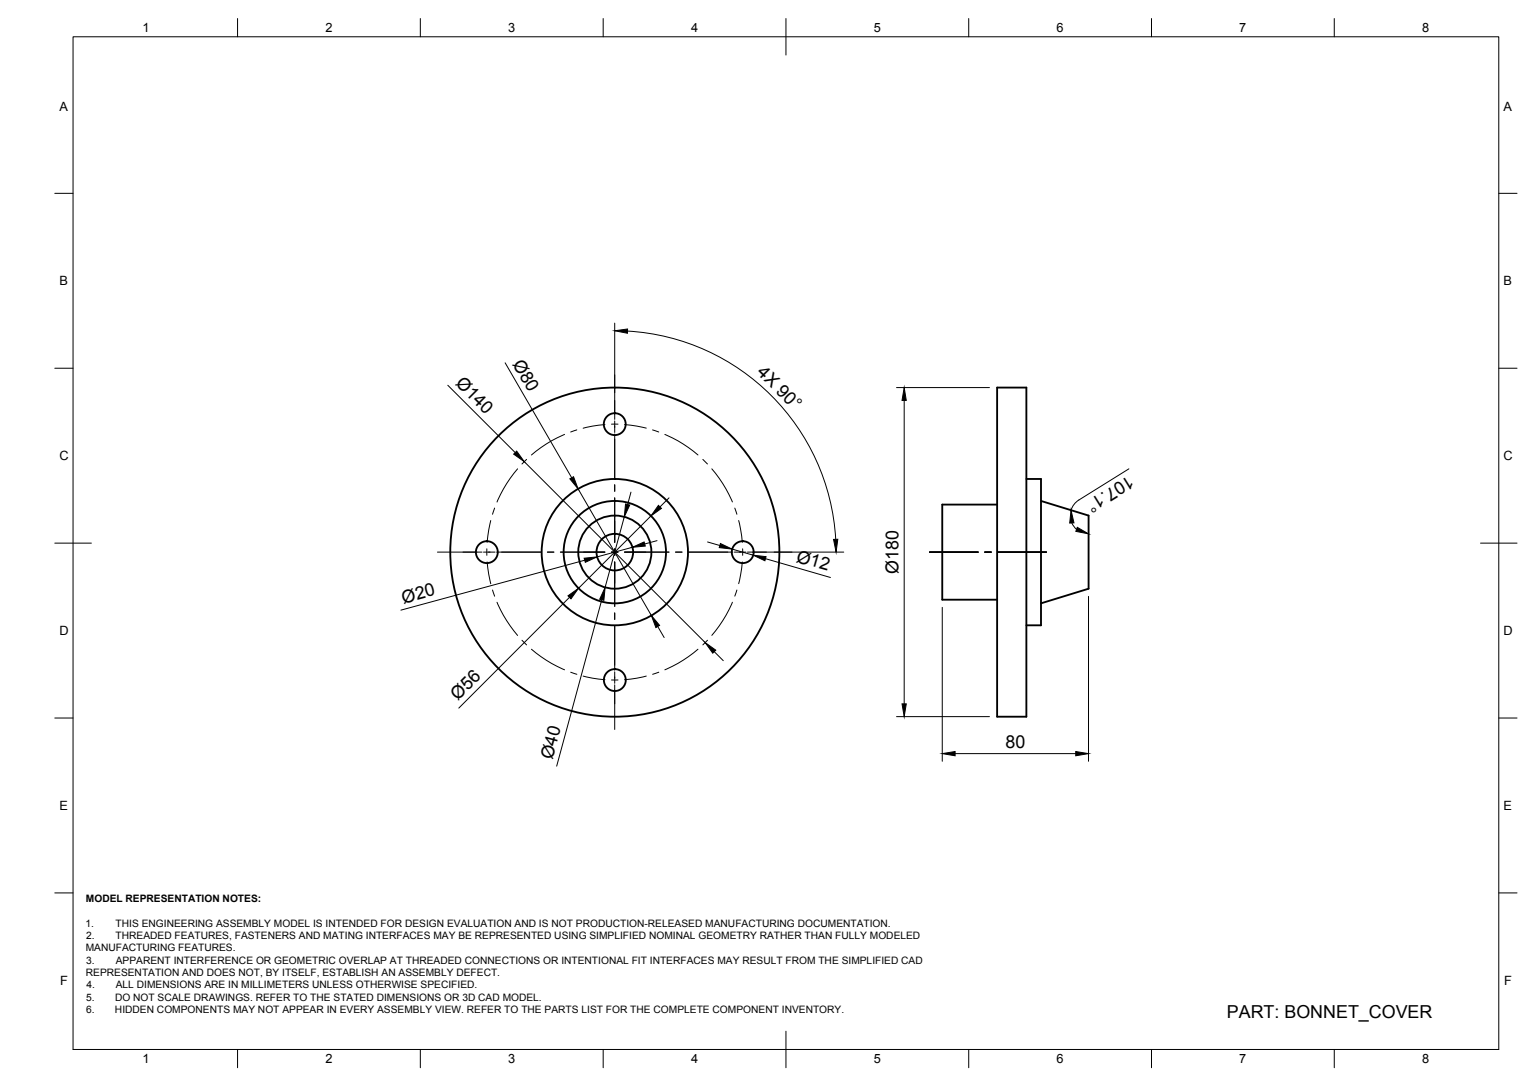
ISO-10303-21;
HEADER;
/* Generated by software containing ST-Developer
 * from STEP Tools, Inc. (www.steptools.com) 
 */

FILE_DESCRIPTION(
/* description */ (''),
/* implementation_level */ '2;1');

FILE_NAME(
/* name */ 'BONNET_COVER.step',
/* time_stamp */ '2026-10-04T02:10:06-07:00',
/* author */ (''),
/* organization */ (''),
/* preprocessor_version */ 'ST-DEVELOPER v20.2',
/* originating_system */ 'Autodesk Translation Framework v15.15.0.0',
/* authorisation */ '');

FILE_SCHEMA (('AUTOMOTIVE_DESIGN { 1 0 10303 214 3 1 1 }'));
ENDSEC;

DATA;
#10=MECHANICAL_DESIGN_GEOMETRIC_PRESENTATION_REPRESENTATION('',(#146),#9668);
#124=SHAPE_REPRESENTATION_RELATIONSHIP('SRR','None',#9717,#135);
#135=ADVANCED_BREP_SHAPE_REPRESENTATION('',(#157),#9662);
#146=STYLED_ITEM('',(#9775),#157);
#157=MANIFOLD_SOLID_BREP('Body1',#3886);
#173=CONICAL_SURFACE('',#4247,18.,1.1071487177941);
#174=CONICAL_SURFACE('',#4254,19.9999999999999,0.298498931586182);
#241=FACE_BOUND('',#1184,.T.);
#242=FACE_BOUND('',#1189,.T.);
#243=FACE_BOUND('',#1192,.T.);
#244=FACE_BOUND('',#1195,.T.);
#245=FACE_BOUND('',#1196,.T.);
#246=FACE_BOUND('',#1197,.T.);
#247=FACE_BOUND('',#1198,.T.);
#248=FACE_BOUND('',#1199,.T.);
#249=FACE_BOUND('',#1202,.T.);
#250=FACE_BOUND('',#1203,.T.);
#251=FACE_BOUND('',#1204,.T.);
#252=FACE_BOUND('',#1205,.T.);
#253=FACE_BOUND('',#1206,.T.);
#315=PLANE('',#4241);
#316=PLANE('',#4252);
#317=PLANE('',#4256);
#318=PLANE('',#4260);
#319=PLANE('',#4268);
#473=LINE('',#6782,#664);
#474=LINE('',#6791,#665);
#475=LINE('',#6794,#666);
#476=LINE('',#6802,#667);
#477=LINE('',#6808,#668);
#478=LINE('',#6823,#669);
#479=LINE('',#6837,#670);
#480=LINE('',#6839,#671);
#481=LINE('',#6841,#672);
#482=LINE('',#6843,#673);
#483=LINE('',#6845,#674);
#664=VECTOR('',#5033,18.0000000000001);
#665=VECTOR('',#5044,18.);
#666=VECTOR('',#5047,9.99999999999995);
#667=VECTOR('',#5058,19.9999999999999);
#668=VECTOR('',#5065,40.);
#669=VECTOR('',#5082,89.999999999998);
#670=VECTOR('',#5099,25.999999999998);
#671=VECTOR('',#5102,6.);
#672=VECTOR('',#5105,6.);
#673=VECTOR('',#5108,6.);
#674=VECTOR('',#5111,6.);
#792=CYLINDRICAL_SURFACE('',#4244,18.0000000000001);
#793=CYLINDRICAL_SURFACE('',#4250,9.99999999999995);
#794=CYLINDRICAL_SURFACE('',#4258,40.);
#795=CYLINDRICAL_SURFACE('',#4266,89.999999999998);
#796=CYLINDRICAL_SURFACE('',#4274,25.999999999998);
#797=CYLINDRICAL_SURFACE('',#4275,6.);
#798=CYLINDRICAL_SURFACE('',#4276,6.);
#799=CYLINDRICAL_SURFACE('',#4277,6.);
#800=CYLINDRICAL_SURFACE('',#4278,6.);
#914=FACE_OUTER_BOUND('',#1183,.T.);
#915=FACE_OUTER_BOUND('',#1185,.T.);
#916=FACE_OUTER_BOUND('',#1186,.T.);
#917=FACE_OUTER_BOUND('',#1187,.T.);
#918=FACE_OUTER_BOUND('',#1188,.T.);
#919=FACE_OUTER_BOUND('',#1190,.T.);
#920=FACE_OUTER_BOUND('',#1191,.T.);
#921=FACE_OUTER_BOUND('',#1193,.T.);
#922=FACE_OUTER_BOUND('',#1194,.T.);
#923=FACE_OUTER_BOUND('',#1200,.T.);
#924=FACE_OUTER_BOUND('',#1201,.T.);
#925=FACE_OUTER_BOUND('',#1207,.T.);
#926=FACE_OUTER_BOUND('',#1208,.T.);
#927=FACE_OUTER_BOUND('',#1209,.T.);
#928=FACE_OUTER_BOUND('',#1210,.T.);
#929=FACE_OUTER_BOUND('',#1211,.T.);
#1183=EDGE_LOOP('',(#3053));
#1184=EDGE_LOOP('',(#3054));
#1185=EDGE_LOOP('',(#3055,#3056,#3057,#3058,#3059));
#1186=EDGE_LOOP('',(#3060,#3061,#3062,#3063,#3064,#3065));
#1187=EDGE_LOOP('',(#3066,#3067,#3068,#3069,#3070));
#1188=EDGE_LOOP('',(#3071));
#1189=EDGE_LOOP('',(#3072));
#1190=EDGE_LOOP('',(#3073,#3074,#3075,#3076));
#1191=EDGE_LOOP('',(#3077));
#1192=EDGE_LOOP('',(#3078));
#1193=EDGE_LOOP('',(#3079,#3080,#3081,#3082));
#1194=EDGE_LOOP('',(#3083));
#1195=EDGE_LOOP('',(#3084));
#1196=EDGE_LOOP('',(#3085));
#1197=EDGE_LOOP('',(#3086));
#1198=EDGE_LOOP('',(#3087));
#1199=EDGE_LOOP('',(#3088));
#1200=EDGE_LOOP('',(#3089,#3090,#3091,#3092));
#1201=EDGE_LOOP('',(#3093));
#1202=EDGE_LOOP('',(#3094));
#1203=EDGE_LOOP('',(#3095));
#1204=EDGE_LOOP('',(#3096));
#1205=EDGE_LOOP('',(#3097));
#1206=EDGE_LOOP('',(#3098));
#1207=EDGE_LOOP('',(#3099,#3100,#3101,#3102));
#1208=EDGE_LOOP('',(#3103,#3104,#3105,#3106));
#1209=EDGE_LOOP('',(#3107,#3108,#3109,#3110));
#1210=EDGE_LOOP('',(#3111,#3112,#3113,#3114));
#1211=EDGE_LOOP('',(#3115,#3116,#3117,#3118));
#1543=CIRCLE('',#4242,25.999999999998);
#1544=CIRCLE('',#4243,18.0000000000002);
#1545=CIRCLE('',#4245,18.);
#1546=CIRCLE('',#4246,18.);
#1547=CIRCLE('',#4248,10.);
#1548=CIRCLE('',#4249,10.);
#1549=CIRCLE('',#4251,9.9999999999999);
#1550=CIRCLE('',#4253,19.9999999999999);
#1551=CIRCLE('',#4255,28.);
#1552=CIRCLE('',#4257,40.);
#1553=CIRCLE('',#4259,40.);
#1554=CIRCLE('',#4261,89.999999999998);
#1555=CIRCLE('',#4262,6.);
#1556=CIRCLE('',#4263,6.);
#1557=CIRCLE('',#4264,6.);
#1558=CIRCLE('',#4265,6.);
#1559=CIRCLE('',#4267,89.999999999998);
#1560=CIRCLE('',#4269,6.);
#1561=CIRCLE('',#4270,6.);
#1562=CIRCLE('',#4271,6.);
#1563=CIRCLE('',#4272,6.);
#1564=CIRCLE('',#4273,25.9999999999979);
#1809=VERTEX_POINT('',#6776);
#1810=VERTEX_POINT('',#6778);
#1811=VERTEX_POINT('',#6781);
#1812=VERTEX_POINT('',#6783);
#1813=VERTEX_POINT('',#6787);
#1814=VERTEX_POINT('',#6788);
#1815=VERTEX_POINT('',#6793);
#1816=VERTEX_POINT('',#6797);
#1817=VERTEX_POINT('',#6800);
#1818=VERTEX_POINT('',#6804);
#1819=VERTEX_POINT('',#6807);
#1820=VERTEX_POINT('',#6811);
#1821=VERTEX_POINT('',#6813);
#1822=VERTEX_POINT('',#6815);
#1823=VERTEX_POINT('',#6817);
#1824=VERTEX_POINT('',#6819);
#1825=VERTEX_POINT('',#6822);
#1826=VERTEX_POINT('',#6826);
#1827=VERTEX_POINT('',#6828);
#1828=VERTEX_POINT('',#6830);
#1829=VERTEX_POINT('',#6832);
#1830=VERTEX_POINT('',#6834);
#2250=EDGE_CURVE('',#1809,#1809,#1543,.T.);
#2251=EDGE_CURVE('',#1810,#1810,#1544,.T.);
#2252=EDGE_CURVE('',#1810,#1811,#473,.T.);
#2253=EDGE_CURVE('',#1811,#1812,#1545,.T.);
#2254=EDGE_CURVE('',#1812,#1811,#1546,.T.);
#2255=EDGE_CURVE('',#1813,#1814,#1547,.T.);
#2256=EDGE_CURVE('',#1814,#1813,#1548,.T.);
#2257=EDGE_CURVE('',#1813,#1812,#474,.T.);
#2258=EDGE_CURVE('',#1814,#1815,#475,.T.);
#2259=EDGE_CURVE('',#1815,#1815,#1549,.T.);
#2260=EDGE_CURVE('',#1816,#1816,#1550,.T.);
#2261=EDGE_CURVE('',#1817,#1817,#1551,.T.);
#2262=EDGE_CURVE('',#1817,#1816,#476,.T.);
#2263=EDGE_CURVE('',#1818,#1818,#1552,.T.);
#2264=EDGE_CURVE('',#1818,#1819,#477,.T.);
#2265=EDGE_CURVE('',#1819,#1819,#1553,.T.);
#2266=EDGE_CURVE('',#1820,#1820,#1554,.T.);
#2267=EDGE_CURVE('',#1821,#1821,#1555,.T.);
#2268=EDGE_CURVE('',#1822,#1822,#1556,.T.);
#2269=EDGE_CURVE('',#1823,#1823,#1557,.T.);
#2270=EDGE_CURVE('',#1824,#1824,#1558,.T.);
#2271=EDGE_CURVE('',#1820,#1825,#478,.T.);
#2272=EDGE_CURVE('',#1825,#1825,#1559,.T.);
#2273=EDGE_CURVE('',#1826,#1826,#1560,.T.);
#2274=EDGE_CURVE('',#1827,#1827,#1561,.T.);
#2275=EDGE_CURVE('',#1828,#1828,#1562,.T.);
#2276=EDGE_CURVE('',#1829,#1829,#1563,.T.);
#2277=EDGE_CURVE('',#1830,#1830,#1564,.T.);
#2278=EDGE_CURVE('',#1830,#1809,#479,.T.);
#2279=EDGE_CURVE('',#1824,#1829,#480,.T.);
#2280=EDGE_CURVE('',#1823,#1828,#481,.T.);
#2281=EDGE_CURVE('',#1822,#1827,#482,.T.);
#2282=EDGE_CURVE('',#1821,#1826,#483,.T.);
#3053=ORIENTED_EDGE('',*,*,#2250,.F.);
#3054=ORIENTED_EDGE('',*,*,#2251,.T.);
#3055=ORIENTED_EDGE('',*,*,#2251,.F.);
#3056=ORIENTED_EDGE('',*,*,#2252,.T.);
#3057=ORIENTED_EDGE('',*,*,#2253,.T.);
#3058=ORIENTED_EDGE('',*,*,#2254,.T.);
#3059=ORIENTED_EDGE('',*,*,#2252,.F.);
#3060=ORIENTED_EDGE('',*,*,#2255,.T.);
#3061=ORIENTED_EDGE('',*,*,#2256,.T.);
#3062=ORIENTED_EDGE('',*,*,#2257,.T.);
#3063=ORIENTED_EDGE('',*,*,#2253,.F.);
#3064=ORIENTED_EDGE('',*,*,#2254,.F.);
#3065=ORIENTED_EDGE('',*,*,#2257,.F.);
#3066=ORIENTED_EDGE('',*,*,#2255,.F.);
#3067=ORIENTED_EDGE('',*,*,#2256,.F.);
#3068=ORIENTED_EDGE('',*,*,#2258,.T.);
#3069=ORIENTED_EDGE('',*,*,#2259,.T.);
#3070=ORIENTED_EDGE('',*,*,#2258,.F.);
#3071=ORIENTED_EDGE('',*,*,#2260,.T.);
#3072=ORIENTED_EDGE('',*,*,#2259,.F.);
#3073=ORIENTED_EDGE('',*,*,#2261,.T.);
#3074=ORIENTED_EDGE('',*,*,#2262,.T.);
#3075=ORIENTED_EDGE('',*,*,#2260,.F.);
#3076=ORIENTED_EDGE('',*,*,#2262,.F.);
#3077=ORIENTED_EDGE('',*,*,#2263,.T.);
#3078=ORIENTED_EDGE('',*,*,#2261,.F.);
#3079=ORIENTED_EDGE('',*,*,#2263,.F.);
#3080=ORIENTED_EDGE('',*,*,#2264,.T.);
#3081=ORIENTED_EDGE('',*,*,#2265,.T.);
#3082=ORIENTED_EDGE('',*,*,#2264,.F.);
#3083=ORIENTED_EDGE('',*,*,#2266,.T.);
#3084=ORIENTED_EDGE('',*,*,#2265,.F.);
#3085=ORIENTED_EDGE('',*,*,#2267,.F.);
#3086=ORIENTED_EDGE('',*,*,#2268,.F.);
#3087=ORIENTED_EDGE('',*,*,#2269,.F.);
#3088=ORIENTED_EDGE('',*,*,#2270,.F.);
#3089=ORIENTED_EDGE('',*,*,#2266,.F.);
#3090=ORIENTED_EDGE('',*,*,#2271,.T.);
#3091=ORIENTED_EDGE('',*,*,#2272,.T.);
#3092=ORIENTED_EDGE('',*,*,#2271,.F.);
#3093=ORIENTED_EDGE('',*,*,#2272,.F.);
#3094=ORIENTED_EDGE('',*,*,#2273,.F.);
#3095=ORIENTED_EDGE('',*,*,#2274,.F.);
#3096=ORIENTED_EDGE('',*,*,#2275,.F.);
#3097=ORIENTED_EDGE('',*,*,#2276,.F.);
#3098=ORIENTED_EDGE('',*,*,#2277,.T.);
#3099=ORIENTED_EDGE('',*,*,#2277,.F.);
#3100=ORIENTED_EDGE('',*,*,#2278,.T.);
#3101=ORIENTED_EDGE('',*,*,#2250,.T.);
#3102=ORIENTED_EDGE('',*,*,#2278,.F.);
#3103=ORIENTED_EDGE('',*,*,#2270,.T.);
#3104=ORIENTED_EDGE('',*,*,#2279,.T.);
#3105=ORIENTED_EDGE('',*,*,#2276,.T.);
#3106=ORIENTED_EDGE('',*,*,#2279,.F.);
#3107=ORIENTED_EDGE('',*,*,#2269,.T.);
#3108=ORIENTED_EDGE('',*,*,#2280,.T.);
#3109=ORIENTED_EDGE('',*,*,#2275,.T.);
#3110=ORIENTED_EDGE('',*,*,#2280,.F.);
#3111=ORIENTED_EDGE('',*,*,#2268,.T.);
#3112=ORIENTED_EDGE('',*,*,#2281,.T.);
#3113=ORIENTED_EDGE('',*,*,#2274,.T.);
#3114=ORIENTED_EDGE('',*,*,#2281,.F.);
#3115=ORIENTED_EDGE('',*,*,#2267,.T.);
#3116=ORIENTED_EDGE('',*,*,#2282,.T.);
#3117=ORIENTED_EDGE('',*,*,#2273,.T.);
#3118=ORIENTED_EDGE('',*,*,#2282,.F.);
#3762=ADVANCED_FACE('',(#914,#241),#315,.T.);
#3763=ADVANCED_FACE('',(#915),#792,.F.);
#3764=ADVANCED_FACE('',(#916),#173,.F.);
#3765=ADVANCED_FACE('',(#917),#793,.F.);
#3766=ADVANCED_FACE('',(#918,#242),#316,.T.);
#3767=ADVANCED_FACE('',(#919),#174,.T.);
#3768=ADVANCED_FACE('',(#920,#243),#317,.T.);
#3769=ADVANCED_FACE('',(#921),#794,.T.);
#3770=ADVANCED_FACE('',(#922,#244,#245,#246,#247,#248),#318,.T.);
#3771=ADVANCED_FACE('',(#923),#795,.T.);
#3772=ADVANCED_FACE('',(#924,#249,#250,#251,#252,#253),#319,.T.);
#3773=ADVANCED_FACE('',(#925),#796,.T.);
#3774=ADVANCED_FACE('',(#926),#797,.F.);
#3775=ADVANCED_FACE('',(#927),#798,.F.);
#3776=ADVANCED_FACE('',(#928),#799,.F.);
#3777=ADVANCED_FACE('',(#929),#800,.F.);
#3886=CLOSED_SHELL('',(#3762,#3763,#3764,#3765,#3766,#3767,#3768,#3769,
#3770,#3771,#3772,#3773,#3774,#3775,#3776,#3777));
#4240=AXIS2_PLACEMENT_3D('',#6774,#5023,#5024);
#4241=AXIS2_PLACEMENT_3D('',#6775,#5025,#5026);
#4242=AXIS2_PLACEMENT_3D('',#6777,#5027,#5028);
#4243=AXIS2_PLACEMENT_3D('',#6779,#5029,#5030);
#4244=AXIS2_PLACEMENT_3D('',#6780,#5031,#5032);
#4245=AXIS2_PLACEMENT_3D('',#6784,#5034,#5035);
#4246=AXIS2_PLACEMENT_3D('',#6785,#5036,#5037);
#4247=AXIS2_PLACEMENT_3D('',#6786,#5038,#5039);
#4248=AXIS2_PLACEMENT_3D('',#6789,#5040,#5041);
#4249=AXIS2_PLACEMENT_3D('',#6790,#5042,#5043);
#4250=AXIS2_PLACEMENT_3D('',#6792,#5045,#5046);
#4251=AXIS2_PLACEMENT_3D('',#6795,#5048,#5049);
#4252=AXIS2_PLACEMENT_3D('',#6796,#5050,#5051);
#4253=AXIS2_PLACEMENT_3D('',#6798,#5052,#5053);
#4254=AXIS2_PLACEMENT_3D('',#6799,#5054,#5055);
#4255=AXIS2_PLACEMENT_3D('',#6801,#5056,#5057);
#4256=AXIS2_PLACEMENT_3D('',#6803,#5059,#5060);
#4257=AXIS2_PLACEMENT_3D('',#6805,#5061,#5062);
#4258=AXIS2_PLACEMENT_3D('',#6806,#5063,#5064);
#4259=AXIS2_PLACEMENT_3D('',#6809,#5066,#5067);
#4260=AXIS2_PLACEMENT_3D('',#6810,#5068,#5069);
#4261=AXIS2_PLACEMENT_3D('',#6812,#5070,#5071);
#4262=AXIS2_PLACEMENT_3D('',#6814,#5072,#5073);
#4263=AXIS2_PLACEMENT_3D('',#6816,#5074,#5075);
#4264=AXIS2_PLACEMENT_3D('',#6818,#5076,#5077);
#4265=AXIS2_PLACEMENT_3D('',#6820,#5078,#5079);
#4266=AXIS2_PLACEMENT_3D('',#6821,#5080,#5081);
#4267=AXIS2_PLACEMENT_3D('',#6824,#5083,#5084);
#4268=AXIS2_PLACEMENT_3D('',#6825,#5085,#5086);
#4269=AXIS2_PLACEMENT_3D('',#6827,#5087,#5088);
#4270=AXIS2_PLACEMENT_3D('',#6829,#5089,#5090);
#4271=AXIS2_PLACEMENT_3D('',#6831,#5091,#5092);
#4272=AXIS2_PLACEMENT_3D('',#6833,#5093,#5094);
#4273=AXIS2_PLACEMENT_3D('',#6835,#5095,#5096);
#4274=AXIS2_PLACEMENT_3D('',#6836,#5097,#5098);
#4275=AXIS2_PLACEMENT_3D('',#6838,#5100,#5101);
#4276=AXIS2_PLACEMENT_3D('',#6840,#5103,#5104);
#4277=AXIS2_PLACEMENT_3D('',#6842,#5106,#5107);
#4278=AXIS2_PLACEMENT_3D('',#6844,#5109,#5110);
#5023=DIRECTION('axis',(0.,0.,1.));
#5024=DIRECTION('refdir',(1.,0.,0.));
#5025=DIRECTION('center_axis',(-3.43024899888577E-15,1.,0.));
#5026=DIRECTION('ref_axis',(0.,0.,1.));
#5027=DIRECTION('center_axis',(3.43024899888577E-15,-1.,0.));
#5028=DIRECTION('ref_axis',(1.,3.43024899888577E-15,0.));
#5029=DIRECTION('center_axis',(3.43024899888577E-15,-1.,0.));
#5030=DIRECTION('ref_axis',(1.,3.43024899888577E-15,0.));
#5031=DIRECTION('center_axis',(3.43024899888577E-15,-1.,0.));
#5032=DIRECTION('ref_axis',(1.,3.43024899888577E-15,0.));
#5033=DIRECTION('',(3.43024899888577E-15,-1.,0.));
#5034=DIRECTION('center_axis',(3.43024899888577E-15,-1.,0.));
#5035=DIRECTION('ref_axis',(1.,3.43024899888577E-15,0.));
#5036=DIRECTION('center_axis',(3.43024899888577E-15,-1.,0.));
#5037=DIRECTION('ref_axis',(1.,3.43024899888577E-15,0.));
#5038=DIRECTION('center_axis',(-3.43024899888577E-15,1.,0.));
#5039=DIRECTION('ref_axis',(-1.,-3.43024899888577E-15,0.));
#5040=DIRECTION('center_axis',(3.43024899888577E-15,-1.,0.));
#5041=DIRECTION('ref_axis',(1.,3.43024899888577E-15,0.));
#5042=DIRECTION('center_axis',(3.43024899888577E-15,-1.,0.));
#5043=DIRECTION('ref_axis',(1.,3.43024899888577E-15,0.));
#5044=DIRECTION('',(0.89442719099992,0.44721359549995,-1.09535739652841E-16));
#5045=DIRECTION('center_axis',(3.43024899888577E-15,-1.,0.));
#5046=DIRECTION('ref_axis',(1.,3.43024899888577E-15,0.));
#5047=DIRECTION('',(3.43024899888577E-15,-1.,0.));
#5048=DIRECTION('center_axis',(3.43024899888577E-15,-1.,0.));
#5049=DIRECTION('ref_axis',(1.,3.43024899888577E-15,0.));
#5050=DIRECTION('center_axis',(3.43024899888577E-15,-1.,0.));
#5051=DIRECTION('ref_axis',(0.,0.,-1.));
#5052=DIRECTION('center_axis',(3.43024899888577E-15,-1.,0.));
#5053=DIRECTION('ref_axis',(1.,3.43024899888577E-15,0.));
#5054=DIRECTION('center_axis',(-3.43024899888577E-15,1.,0.));
#5055=DIRECTION('ref_axis',(-1.,-3.43024899888577E-15,0.));
#5056=DIRECTION('center_axis',(3.43024899888577E-15,-1.,0.));
#5057=DIRECTION('ref_axis',(1.,3.43024899888577E-15,0.));
#5058=DIRECTION('',(-0.294085848837523,-0.95577900872195,3.60151293453408E-17));
#5059=DIRECTION('center_axis',(3.43024899888577E-15,-1.,0.));
#5060=DIRECTION('ref_axis',(0.,0.,-1.));
#5061=DIRECTION('center_axis',(3.43024899888577E-15,-1.,0.));
#5062=DIRECTION('ref_axis',(1.,3.43024899888577E-15,0.));
#5063=DIRECTION('center_axis',(3.43024899888577E-15,-1.,0.));
#5064=DIRECTION('ref_axis',(1.,3.43024899888577E-15,0.));
#5065=DIRECTION('',(-3.43024899888577E-15,1.,0.));
#5066=DIRECTION('center_axis',(3.43024899888577E-15,-1.,0.));
#5067=DIRECTION('ref_axis',(1.,3.43024899888577E-15,0.));
#5068=DIRECTION('center_axis',(3.43024899888577E-15,-1.,0.));
#5069=DIRECTION('ref_axis',(0.,0.,-1.));
#5070=DIRECTION('center_axis',(3.43024899888577E-15,-1.,0.));
#5071=DIRECTION('ref_axis',(1.,3.43024899888577E-15,0.));
#5072=DIRECTION('center_axis',(3.43024899888577E-15,-1.,0.));
#5073=DIRECTION('ref_axis',(1.,3.43024899888577E-15,0.));
#5074=DIRECTION('center_axis',(3.43024899888577E-15,-1.,0.));
#5075=DIRECTION('ref_axis',(1.,3.43024899888577E-15,0.));
#5076=DIRECTION('center_axis',(3.43024899888577E-15,-1.,0.));
#5077=DIRECTION('ref_axis',(1.,3.43024899888577E-15,0.));
#5078=DIRECTION('center_axis',(3.43024899888577E-15,-1.,0.));
#5079=DIRECTION('ref_axis',(1.,3.43024899888577E-15,0.));
#5080=DIRECTION('center_axis',(3.43024899888577E-15,-1.,0.));
#5081=DIRECTION('ref_axis',(1.,3.43024899888577E-15,0.));
#5082=DIRECTION('',(-3.43024899888577E-15,1.,0.));
#5083=DIRECTION('center_axis',(3.43024899888577E-15,-1.,0.));
#5084=DIRECTION('ref_axis',(1.,3.43024899888577E-15,0.));
#5085=DIRECTION('center_axis',(-3.43024899888577E-15,1.,0.));
#5086=DIRECTION('ref_axis',(0.,0.,1.));
#5087=DIRECTION('center_axis',(-3.43024899888577E-15,1.,5.91645678915759E-30));
#5088=DIRECTION('ref_axis',(3.49148133884313E-15,1.81438008200833E-29,-1.));
#5089=DIRECTION('center_axis',(-3.43024899888578E-15,1.,0.));
#5090=DIRECTION('ref_axis',(1.,3.43024899888578E-15,0.));
#5091=DIRECTION('center_axis',(-3.43024899888577E-15,1.,-5.91645678915759E-30));
#5092=DIRECTION('ref_axis',(-1.04744440165294E-14,-2.99767143983984E-29,
1.));
#5093=DIRECTION('center_axis',(-3.43024899888577E-15,1.,0.));
#5094=DIRECTION('ref_axis',(-1.,-3.43024899888577E-15,0.));
#5095=DIRECTION('center_axis',(3.43024899888577E-15,-1.,0.));
#5096=DIRECTION('ref_axis',(1.,3.43024899888577E-15,0.));
#5097=DIRECTION('center_axis',(3.43024899888577E-15,-1.,0.));
#5098=DIRECTION('ref_axis',(1.,3.43024899888577E-15,0.));
#5099=DIRECTION('',(-3.43024899888577E-15,1.,0.));
#5100=DIRECTION('center_axis',(-3.43024899888577E-15,1.,0.));
#5101=DIRECTION('ref_axis',(-1.,-3.43024899888577E-15,0.));
#5102=DIRECTION('',(-3.43024899888577E-15,1.,0.));
#5103=DIRECTION('center_axis',(-3.43024899888577E-15,1.,-5.91645678915759E-30));
#5104=DIRECTION('ref_axis',(-1.,-3.43024899888577E-15,0.));
#5105=DIRECTION('',(-3.43024899888577E-15,1.,-5.91645678915759E-30));
#5106=DIRECTION('center_axis',(-3.43024899888578E-15,1.,0.));
#5107=DIRECTION('ref_axis',(-1.,-3.43024899888578E-15,0.));
#5108=DIRECTION('',(-3.43024899888578E-15,1.,0.));
#5109=DIRECTION('center_axis',(-3.43024899888577E-15,1.,5.91645678915759E-30));
#5110=DIRECTION('ref_axis',(-1.,-3.43024899888577E-15,0.));
#5111=DIRECTION('',(-3.43024899888577E-15,1.,5.91645678915759E-30));
#6774=CARTESIAN_POINT('',(0.,0.,0.));
#6775=CARTESIAN_POINT('Origin',(25.9999999999979,50.,0.));
#6776=CARTESIAN_POINT('',(-25.9999999999982,49.9999999999998,-3.18408167778287E-15));
#6777=CARTESIAN_POINT('Origin',(-1.71512449944288E-13,49.9999999999998,
0.));
#6778=CARTESIAN_POINT('',(-18.0000000000003,49.9999999999998,-2.20436423846525E-15));
#6779=CARTESIAN_POINT('Origin',(-1.71512449944288E-13,49.9999999999998,
0.));
#6780=CARTESIAN_POINT('Origin',(2.05611259281969E-12,-599.406221964517,
0.));
#6781=CARTESIAN_POINT('',(-18.0000000000001,3.99999999999984,-2.20436423846525E-15));
#6782=CARTESIAN_POINT('',(-17.999999999998,-599.406221964517,-2.20436423846525E-15));
#6783=CARTESIAN_POINT('',(18.,3.99999999999995,0.));
#6784=CARTESIAN_POINT('Origin',(-1.37209959955424E-14,3.99999999999989,
0.));
#6785=CARTESIAN_POINT('Origin',(-1.37209959955424E-14,3.99999999999989,
0.));
#6786=CARTESIAN_POINT('Origin',(-1.37209959955424E-14,3.99999999999989,
0.));
#6787=CARTESIAN_POINT('',(10.,3.43024899888577E-14,0.));
#6788=CARTESIAN_POINT('',(-9.99999999999995,0.,-1.22464679914735E-15));
#6789=CARTESIAN_POINT('Origin',(0.,0.,0.));
#6790=CARTESIAN_POINT('Origin',(0.,0.,0.));
#6791=CARTESIAN_POINT('',(18.,3.99999999999995,-2.20436423846524E-15));
#6792=CARTESIAN_POINT('Origin',(2.05611259281969E-12,-599.406221964517,
0.));
#6793=CARTESIAN_POINT('',(-9.99999999999985,-30.0000000000001,-1.22464679914735E-15));
#6794=CARTESIAN_POINT('',(-9.99999999999789,-599.406221964517,-1.22464679914735E-15));
#6795=CARTESIAN_POINT('Origin',(1.02907469966573E-13,-30.,0.));
#6796=CARTESIAN_POINT('Origin',(10.,-30.,0.));
#6797=CARTESIAN_POINT('',(20.,-30.0000000000001,0.));
#6798=CARTESIAN_POINT('Origin',(1.02907469966574E-13,-30.0000000000001,
0.));
#6799=CARTESIAN_POINT('Origin',(1.02907469966574E-13,-30.0000000000001,
0.));
#6800=CARTESIAN_POINT('',(28.,-4.00000000000002,0.));
#6801=CARTESIAN_POINT('Origin',(1.37209959955436E-14,-4.00000000000011,
0.));
#6802=CARTESIAN_POINT('',(20.,-30.0000000000001,-2.44929359829469E-15));
#6803=CARTESIAN_POINT('Origin',(28.,-4.00000000000002,0.));
#6804=CARTESIAN_POINT('',(-40.,-4.00000000000027,-4.89858719658941E-15));
#6805=CARTESIAN_POINT('Origin',(1.37209959955436E-14,-4.00000000000011,
0.));
#6806=CARTESIAN_POINT('Origin',(2.05611259281969E-12,-599.406221964517,
0.));
#6807=CARTESIAN_POINT('',(-40.,3.99999999999977,-4.89858719658941E-15));
#6808=CARTESIAN_POINT('',(-39.9999999999979,-599.406221964517,-4.89858719658941E-15));
#6809=CARTESIAN_POINT('Origin',(-1.37209959955424E-14,3.99999999999989,
0.));
#6810=CARTESIAN_POINT('Origin',(40.,3.99999999999992,0.));
#6811=CARTESIAN_POINT('',(-89.999999999998,3.99999999999935,-1.10218211923259E-14));
#6812=CARTESIAN_POINT('Origin',(-1.37209959955416E-14,3.99999999999967,
0.));
#6813=CARTESIAN_POINT('',(-64.,3.99999999999956,-2.44403693719019E-13));
#6814=CARTESIAN_POINT('Origin',(-70.,3.99999999999954,-2.44403693719019E-13));
#6815=CARTESIAN_POINT('',(5.99999999999999,3.9999999999998,-70.));
#6816=CARTESIAN_POINT('Origin',(-1.37209959955424E-14,3.99999999999978,
-70.));
#6817=CARTESIAN_POINT('',(76.,4.00000000000004,7.33211081157058E-13));
#6818=CARTESIAN_POINT('Origin',(70.,4.00000000000002,7.33211081157058E-13));
#6819=CARTESIAN_POINT('',(5.99999999999999,3.9999999999998,70.));
#6820=CARTESIAN_POINT('Origin',(-1.37209959955423E-14,3.99999999999978,
70.));
#6821=CARTESIAN_POINT('Origin',(2.05611259281969E-12,-599.406221964517,
0.));
#6822=CARTESIAN_POINT('',(-89.999999999998,19.9999999999994,-1.10218211923259E-14));
#6823=CARTESIAN_POINT('',(-89.9999999999959,-599.406221964518,-1.10218211923259E-14));
#6824=CARTESIAN_POINT('Origin',(-6.86049799777142E-14,19.9999999999997,
0.));
#6825=CARTESIAN_POINT('Origin',(89.9999999999979,20.0000000000001,0.));
#6826=CARTESIAN_POINT('',(-64.0000000000001,19.9999999999996,-2.45138481798508E-13));
#6827=CARTESIAN_POINT('Origin',(-70.0000000000001,19.9999999999996,-2.44403693719019E-13));
#6828=CARTESIAN_POINT('',(5.99999999999993,19.9999999999998,-70.));
#6829=CARTESIAN_POINT('Origin',(-6.86049799777149E-14,19.9999999999998,
-70.));
#6830=CARTESIAN_POINT('',(76.,20.0000000000001,7.3247629307757E-13));
#6831=CARTESIAN_POINT('Origin',(69.9999999999999,20.,7.33211081157058E-13));
#6832=CARTESIAN_POINT('',(5.99999999999993,19.9999999999998,70.));
#6833=CARTESIAN_POINT('Origin',(-6.86049799777146E-14,19.9999999999998,
70.));
#6834=CARTESIAN_POINT('',(-25.9999999999981,19.9999999999998,-3.18408167778287E-15));
#6835=CARTESIAN_POINT('Origin',(-6.86049799777149E-14,19.9999999999999,
0.));
#6836=CARTESIAN_POINT('Origin',(2.05611259281969E-12,-599.406221964517,
0.));
#6837=CARTESIAN_POINT('',(-25.9999999999959,-599.406221964517,-3.18408167778287E-15));
#6838=CARTESIAN_POINT('Origin',(1.02907469966574E-13,-30.0000000000004,
70.));
#6839=CARTESIAN_POINT('',(6.0000000000001,-30.0000000000004,70.));
#6840=CARTESIAN_POINT('Origin',(70.0000000000001,-30.0000000000001,7.33211081157058E-13));
#6841=CARTESIAN_POINT('',(76.0000000000001,-30.0000000000001,7.3247629307757E-13));
#6842=CARTESIAN_POINT('Origin',(1.02907469966575E-13,-30.0000000000004,
-70.));
#6843=CARTESIAN_POINT('',(6.0000000000001,-30.0000000000004,-70.));
#6844=CARTESIAN_POINT('Origin',(-69.9999999999999,-30.0000000000006,-2.4440369371902E-13));
#6845=CARTESIAN_POINT('',(-63.9999999999999,-30.0000000000006,-2.45138481798508E-13));
#9649=UNCERTAINTY_MEASURE_WITH_UNIT(LENGTH_MEASURE(0.01),#9669,
'DISTANCE_ACCURACY_VALUE',
'Maximum model space distance between geometric entities at asserted c
onnectivities');
#9655=UNCERTAINTY_MEASURE_WITH_UNIT(LENGTH_MEASURE(0.01),#9669,
'DISTANCE_ACCURACY_VALUE',
'Maximum model space distance between geometric entities at asserted c
onnectivities');
#9662=(
GEOMETRIC_REPRESENTATION_CONTEXT(3)
GLOBAL_UNCERTAINTY_ASSIGNED_CONTEXT((#9649))
GLOBAL_UNIT_ASSIGNED_CONTEXT((#9669,#9671,#9672))
REPRESENTATION_CONTEXT('','3D')
);
#9668=(
GEOMETRIC_REPRESENTATION_CONTEXT(3)
GLOBAL_UNCERTAINTY_ASSIGNED_CONTEXT((#9655))
GLOBAL_UNIT_ASSIGNED_CONTEXT((#9669,#9671,#9672))
REPRESENTATION_CONTEXT('','3D')
);
#9669=(
LENGTH_UNIT()
NAMED_UNIT(*)
SI_UNIT(.MILLI.,.METRE.)
);
#9671=(
NAMED_UNIT(*)
PLANE_ANGLE_UNIT()
SI_UNIT($,.RADIAN.)
);
#9672=(
NAMED_UNIT(*)
SI_UNIT($,.STERADIAN.)
SOLID_ANGLE_UNIT()
);
#9679=SHAPE_DEFINITION_REPRESENTATION(#9691,#9717);
#9691=PRODUCT_DEFINITION_SHAPE('',$,#9730);
#9717=SHAPE_REPRESENTATION('',(#4240),#9662);
#9723=PRODUCT_DEFINITION_CONTEXT('part definition',#9761,'design');
#9730=PRODUCT_DEFINITION('2026-10-04-08-13-48-885','BONNET_COVER',#9742,
#9723);
#9742=PRODUCT_DEFINITION_FORMATION('',$,#9769);
#9761=APPLICATION_CONTEXT(
'Core Data for Automotive Mechanical Design Process');
#9762=PRODUCT_CONTEXT('part definition',#9761,'mechanical');
#9769=PRODUCT('2026-10-04-08-13-48-885','BONNET_COVER','PART',(#9762));
#9775=PRESENTATION_STYLE_ASSIGNMENT((#9776));
#9776=SURFACE_STYLE_USAGE(.BOTH.,#9777);
#9777=SURFACE_SIDE_STYLE('',(#9778));
#9778=SURFACE_STYLE_FILL_AREA(#9779);
#9779=FILL_AREA_STYLE('Steel - Satin',(#9780));
#9780=FILL_AREA_STYLE_COLOUR('Steel - Satin',#9781);
#9781=COLOUR_RGB('Steel - Satin', 0.09019608, 0.27058824, 0.51372549);
ENDSEC;
END-ISO-10303-21;
